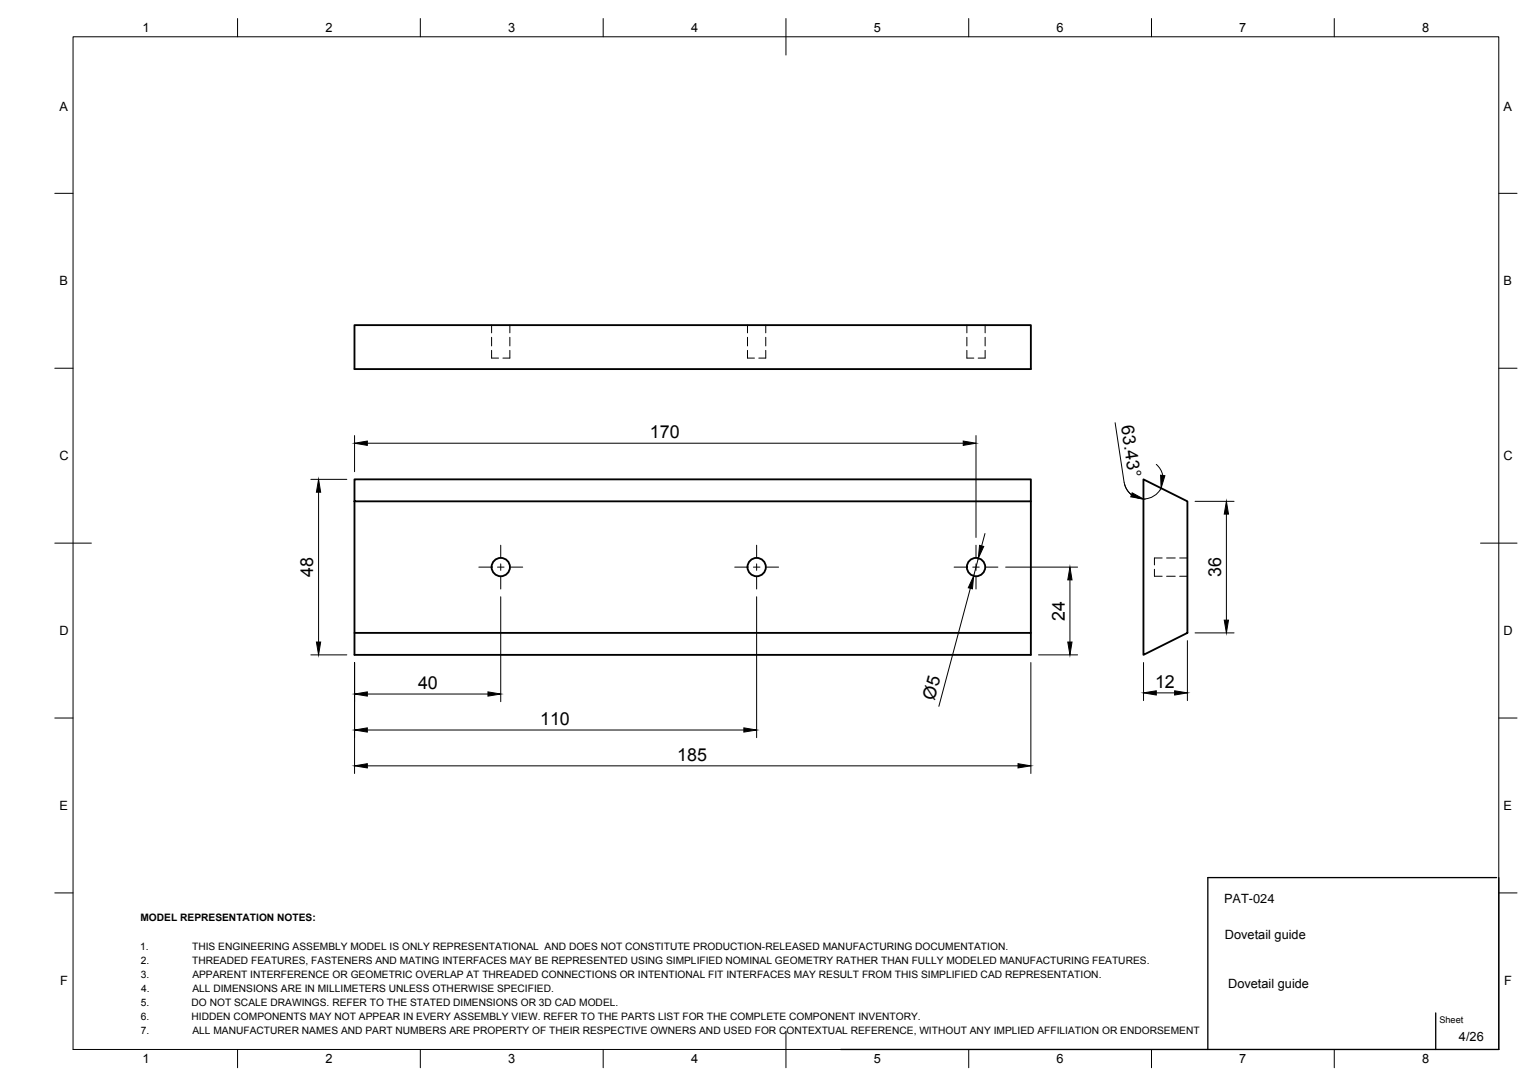
ISO-10303-21;
HEADER;
/* Generated by software containing ST-Developer
 * from STEP Tools, Inc. (www.steptools.com) 
 */

FILE_DESCRIPTION(
/* description */ ('Compact handwheel screw vise'),
/* implementation_level */ '2;1');

FILE_NAME(
/* name */ 'Dovetail guide.step',
/* time_stamp */ '2026-10-29T16:08:22-07:00',
/* author */ (''),
/* organization */ (''),
/* preprocessor_version */ 'ST-DEVELOPER v20.2',
/* originating_system */ 'Autodesk Translation Framework v15.17.0.0',
/* authorisation */ '');

FILE_SCHEMA (('AUTOMOTIVE_DESIGN { 1 0 10303 214 3 1 1 }'));
ENDSEC;

DATA;
#10=MECHANICAL_DESIGN_GEOMETRIC_PRESENTATION_REPRESENTATION('',(#645),#25074);
#589=SHAPE_REPRESENTATION_RELATIONSHIP('SRR','None',#25197,#617);
#617=ADVANCED_BREP_SHAPE_REPRESENTATION('',(#681),#25044);
#645=STYLED_ITEM('',(#25425),#681);
#681=MANIFOLD_SOLID_BREP('Body1',#8053);
#726=FACE_BOUND('',#1518,.T.);
#727=FACE_BOUND('',#1519,.T.);
#728=FACE_BOUND('',#1520,.T.);
#828=PLANE('',#8435);
#829=PLANE('',#8439);
#830=PLANE('',#8443);
#831=PLANE('',#8444);
#832=PLANE('',#8445);
#833=PLANE('',#8446);
#834=PLANE('',#8447);
#835=PLANE('',#8448);
#836=PLANE('',#8449);
#1025=FACE_OUTER_BOUND('',#1509,.T.);
#1026=FACE_OUTER_BOUND('',#1510,.T.);
#1027=FACE_OUTER_BOUND('',#1511,.T.);
#1028=FACE_OUTER_BOUND('',#1512,.T.);
#1029=FACE_OUTER_BOUND('',#1513,.T.);
#1030=FACE_OUTER_BOUND('',#1514,.T.);
#1031=FACE_OUTER_BOUND('',#1515,.T.);
#1032=FACE_OUTER_BOUND('',#1516,.T.);
#1033=FACE_OUTER_BOUND('',#1517,.T.);
#1034=FACE_OUTER_BOUND('',#1521,.T.);
#1035=FACE_OUTER_BOUND('',#1522,.T.);
#1036=FACE_OUTER_BOUND('',#1523,.T.);
#1509=EDGE_LOOP('',(#5225,#5226,#5227,#5228));
#1510=EDGE_LOOP('',(#5229));
#1511=EDGE_LOOP('',(#5230,#5231,#5232,#5233));
#1512=EDGE_LOOP('',(#5234));
#1513=EDGE_LOOP('',(#5235,#5236,#5237,#5238));
#1514=EDGE_LOOP('',(#5239));
#1515=EDGE_LOOP('',(#5240,#5241,#5242,#5243));
#1516=EDGE_LOOP('',(#5244,#5245,#5246,#5247));
#1517=EDGE_LOOP('',(#5248,#5249,#5250,#5251));
#1518=EDGE_LOOP('',(#5252));
#1519=EDGE_LOOP('',(#5253));
#1520=EDGE_LOOP('',(#5254));
#1521=EDGE_LOOP('',(#5255,#5256,#5257,#5258));
#1522=EDGE_LOOP('',(#5259,#5260,#5261,#5262));
#1523=EDGE_LOOP('',(#5263,#5264,#5265,#5266));
#2081=LINE('',#11394,#2589);
#2082=LINE('',#11401,#2590);
#2083=LINE('',#11408,#2591);
#2084=LINE('',#11414,#2592);
#2085=LINE('',#11416,#2593);
#2086=LINE('',#11418,#2594);
#2087=LINE('',#11419,#2595);
#2088=LINE('',#11422,#2596);
#2089=LINE('',#11424,#2597);
#2090=LINE('',#11425,#2598);
#2091=LINE('',#11428,#2599);
#2092=LINE('',#11430,#2600);
#2093=LINE('',#11431,#2601);
#2094=LINE('',#11433,#2602);
#2095=LINE('',#11434,#2603);
#2589=VECTOR('',#9289,0.25);
#2590=VECTOR('',#9298,0.25);
#2591=VECTOR('',#9307,0.25);
#2592=VECTOR('',#9314,1.);
#2593=VECTOR('',#9315,1.);
#2594=VECTOR('',#9316,1.);
#2595=VECTOR('',#9317,1.);
#2596=VECTOR('',#9320,1.);
#2597=VECTOR('',#9321,1.);
#2598=VECTOR('',#9322,1.);
#2599=VECTOR('',#9325,1.);
#2600=VECTOR('',#9326,1.);
#2601=VECTOR('',#9327,1.);
#2602=VECTOR('',#9330,1.);
#2603=VECTOR('',#9331,1.);
#3092=CIRCLE('',#8433,0.25);
#3093=CIRCLE('',#8434,0.25);
#3094=CIRCLE('',#8437,0.25);
#3095=CIRCLE('',#8438,0.25);
#3096=CIRCLE('',#8441,0.25);
#3097=CIRCLE('',#8442,0.25);
#3355=VERTEX_POINT('',#11391);
#3356=VERTEX_POINT('',#11393);
#3357=VERTEX_POINT('',#11398);
#3358=VERTEX_POINT('',#11400);
#3359=VERTEX_POINT('',#11405);
#3360=VERTEX_POINT('',#11407);
#3361=VERTEX_POINT('',#11412);
#3362=VERTEX_POINT('',#11413);
#3363=VERTEX_POINT('',#11415);
#3364=VERTEX_POINT('',#11417);
#3365=VERTEX_POINT('',#11421);
#3366=VERTEX_POINT('',#11423);
#3367=VERTEX_POINT('',#11427);
#3368=VERTEX_POINT('',#11429);
#4099=EDGE_CURVE('',#3355,#3355,#3092,.T.);
#4100=EDGE_CURVE('',#3355,#3356,#2081,.T.);
#4101=EDGE_CURVE('',#3356,#3356,#3093,.T.);
#4102=EDGE_CURVE('',#3357,#3357,#3094,.T.);
#4103=EDGE_CURVE('',#3357,#3358,#2082,.T.);
#4104=EDGE_CURVE('',#3358,#3358,#3095,.T.);
#4105=EDGE_CURVE('',#3359,#3359,#3096,.T.);
#4106=EDGE_CURVE('',#3359,#3360,#2083,.T.);
#4107=EDGE_CURVE('',#3360,#3360,#3097,.T.);
#4108=EDGE_CURVE('',#3361,#3362,#2084,.T.);
#4109=EDGE_CURVE('',#3362,#3363,#2085,.T.);
#4110=EDGE_CURVE('',#3364,#3363,#2086,.T.);
#4111=EDGE_CURVE('',#3361,#3364,#2087,.T.);
#4112=EDGE_CURVE('',#3365,#3361,#2088,.T.);
#4113=EDGE_CURVE('',#3366,#3364,#2089,.T.);
#4114=EDGE_CURVE('',#3365,#3366,#2090,.T.);
#4115=EDGE_CURVE('',#3367,#3365,#2091,.T.);
#4116=EDGE_CURVE('',#3368,#3366,#2092,.T.);
#4117=EDGE_CURVE('',#3367,#3368,#2093,.T.);
#4118=EDGE_CURVE('',#3362,#3367,#2094,.T.);
#4119=EDGE_CURVE('',#3363,#3368,#2095,.T.);
#5225=ORIENTED_EDGE('',*,*,#4099,.F.);
#5226=ORIENTED_EDGE('',*,*,#4100,.T.);
#5227=ORIENTED_EDGE('',*,*,#4101,.T.);
#5228=ORIENTED_EDGE('',*,*,#4100,.F.);
#5229=ORIENTED_EDGE('',*,*,#4101,.F.);
#5230=ORIENTED_EDGE('',*,*,#4102,.F.);
#5231=ORIENTED_EDGE('',*,*,#4103,.T.);
#5232=ORIENTED_EDGE('',*,*,#4104,.T.);
#5233=ORIENTED_EDGE('',*,*,#4103,.F.);
#5234=ORIENTED_EDGE('',*,*,#4104,.F.);
#5235=ORIENTED_EDGE('',*,*,#4105,.F.);
#5236=ORIENTED_EDGE('',*,*,#4106,.T.);
#5237=ORIENTED_EDGE('',*,*,#4107,.T.);
#5238=ORIENTED_EDGE('',*,*,#4106,.F.);
#5239=ORIENTED_EDGE('',*,*,#4107,.F.);
#5240=ORIENTED_EDGE('',*,*,#4108,.T.);
#5241=ORIENTED_EDGE('',*,*,#4109,.T.);
#5242=ORIENTED_EDGE('',*,*,#4110,.F.);
#5243=ORIENTED_EDGE('',*,*,#4111,.F.);
#5244=ORIENTED_EDGE('',*,*,#4112,.T.);
#5245=ORIENTED_EDGE('',*,*,#4111,.T.);
#5246=ORIENTED_EDGE('',*,*,#4113,.F.);
#5247=ORIENTED_EDGE('',*,*,#4114,.F.);
#5248=ORIENTED_EDGE('',*,*,#4115,.T.);
#5249=ORIENTED_EDGE('',*,*,#4114,.T.);
#5250=ORIENTED_EDGE('',*,*,#4116,.F.);
#5251=ORIENTED_EDGE('',*,*,#4117,.F.);
#5252=ORIENTED_EDGE('',*,*,#4099,.T.);
#5253=ORIENTED_EDGE('',*,*,#4102,.T.);
#5254=ORIENTED_EDGE('',*,*,#4105,.T.);
#5255=ORIENTED_EDGE('',*,*,#4118,.T.);
#5256=ORIENTED_EDGE('',*,*,#4117,.T.);
#5257=ORIENTED_EDGE('',*,*,#4119,.F.);
#5258=ORIENTED_EDGE('',*,*,#4109,.F.);
#5259=ORIENTED_EDGE('',*,*,#4119,.T.);
#5260=ORIENTED_EDGE('',*,*,#4116,.T.);
#5261=ORIENTED_EDGE('',*,*,#4113,.T.);
#5262=ORIENTED_EDGE('',*,*,#4110,.T.);
#5263=ORIENTED_EDGE('',*,*,#4118,.F.);
#5264=ORIENTED_EDGE('',*,*,#4108,.F.);
#5265=ORIENTED_EDGE('',*,*,#4112,.F.);
#5266=ORIENTED_EDGE('',*,*,#4115,.F.);
#7352=CYLINDRICAL_SURFACE('',#8432,0.25);
#7353=CYLINDRICAL_SURFACE('',#8436,0.25);
#7354=CYLINDRICAL_SURFACE('',#8440,0.25);
#7595=ADVANCED_FACE('',(#1025),#7352,.F.);
#7596=ADVANCED_FACE('',(#1026),#828,.F.);
#7597=ADVANCED_FACE('',(#1027),#7353,.F.);
#7598=ADVANCED_FACE('',(#1028),#829,.F.);
#7599=ADVANCED_FACE('',(#1029),#7354,.F.);
#7600=ADVANCED_FACE('',(#1030),#830,.F.);
#7601=ADVANCED_FACE('',(#1031),#831,.T.);
#7602=ADVANCED_FACE('',(#1032),#832,.T.);
#7603=ADVANCED_FACE('',(#1033,#726,#727,#728),#833,.T.);
#7604=ADVANCED_FACE('',(#1034),#834,.T.);
#7605=ADVANCED_FACE('',(#1035),#835,.T.);
#7606=ADVANCED_FACE('',(#1036),#836,.F.);
#8053=CLOSED_SHELL('',(#7595,#7596,#7597,#7598,#7599,#7600,#7601,#7602,
#7603,#7604,#7605,#7606));
#8431=AXIS2_PLACEMENT_3D('',#11389,#9283,#9284);
#8432=AXIS2_PLACEMENT_3D('',#11390,#9285,#9286);
#8433=AXIS2_PLACEMENT_3D('',#11392,#9287,#9288);
#8434=AXIS2_PLACEMENT_3D('',#11395,#9290,#9291);
#8435=AXIS2_PLACEMENT_3D('',#11396,#9292,#9293);
#8436=AXIS2_PLACEMENT_3D('',#11397,#9294,#9295);
#8437=AXIS2_PLACEMENT_3D('',#11399,#9296,#9297);
#8438=AXIS2_PLACEMENT_3D('',#11402,#9299,#9300);
#8439=AXIS2_PLACEMENT_3D('',#11403,#9301,#9302);
#8440=AXIS2_PLACEMENT_3D('',#11404,#9303,#9304);
#8441=AXIS2_PLACEMENT_3D('',#11406,#9305,#9306);
#8442=AXIS2_PLACEMENT_3D('',#11409,#9308,#9309);
#8443=AXIS2_PLACEMENT_3D('',#11410,#9310,#9311);
#8444=AXIS2_PLACEMENT_3D('',#11411,#9312,#9313);
#8445=AXIS2_PLACEMENT_3D('',#11420,#9318,#9319);
#8446=AXIS2_PLACEMENT_3D('',#11426,#9323,#9324);
#8447=AXIS2_PLACEMENT_3D('',#11432,#9328,#9329);
#8448=AXIS2_PLACEMENT_3D('',#11435,#9332,#9333);
#8449=AXIS2_PLACEMENT_3D('',#11436,#9334,#9335);
#9283=DIRECTION('axis',(0.,0.,1.));
#9284=DIRECTION('refdir',(1.,0.,0.));
#9285=DIRECTION('center_axis',(0.,0.,1.));
#9286=DIRECTION('ref_axis',(1.,0.,0.));
#9287=DIRECTION('center_axis',(0.,0.,1.));
#9288=DIRECTION('ref_axis',(1.,0.,0.));
#9289=DIRECTION('',(0.,0.,1.));
#9290=DIRECTION('center_axis',(0.,0.,1.));
#9291=DIRECTION('ref_axis',(1.,0.,0.));
#9292=DIRECTION('center_axis',(0.,0.,1.));
#9293=DIRECTION('ref_axis',(1.,0.,0.));
#9294=DIRECTION('center_axis',(0.,0.,1.));
#9295=DIRECTION('ref_axis',(1.,0.,0.));
#9296=DIRECTION('center_axis',(0.,0.,1.));
#9297=DIRECTION('ref_axis',(1.,0.,0.));
#9298=DIRECTION('',(0.,0.,1.));
#9299=DIRECTION('center_axis',(0.,0.,1.));
#9300=DIRECTION('ref_axis',(1.,0.,0.));
#9301=DIRECTION('center_axis',(0.,0.,1.));
#9302=DIRECTION('ref_axis',(1.,0.,0.));
#9303=DIRECTION('center_axis',(0.,0.,1.));
#9304=DIRECTION('ref_axis',(1.,0.,0.));
#9305=DIRECTION('center_axis',(0.,0.,1.));
#9306=DIRECTION('ref_axis',(1.,0.,0.));
#9307=DIRECTION('',(0.,0.,1.));
#9308=DIRECTION('center_axis',(0.,0.,1.));
#9309=DIRECTION('ref_axis',(1.,0.,0.));
#9310=DIRECTION('center_axis',(0.,0.,1.));
#9311=DIRECTION('ref_axis',(1.,0.,0.));
#9312=DIRECTION('center_axis',(0.,0.,1.));
#9313=DIRECTION('ref_axis',(0.,-1.,0.));
#9314=DIRECTION('',(0.,-1.,0.));
#9315=DIRECTION('',(1.,0.,0.));
#9316=DIRECTION('',(0.,-1.,0.));
#9317=DIRECTION('',(1.,0.,0.));
#9318=DIRECTION('center_axis',(0.,0.894427190999916,-0.447213595499958));
#9319=DIRECTION('ref_axis',(0.,0.447213595499958,0.894427190999916));
#9320=DIRECTION('',(0.,0.447213595499958,0.894427190999916));
#9321=DIRECTION('',(0.,0.447213595499958,0.894427190999916));
#9322=DIRECTION('',(1.,0.,0.));
#9323=DIRECTION('center_axis',(0.,0.,-1.));
#9324=DIRECTION('ref_axis',(0.,1.,0.));
#9325=DIRECTION('',(0.,1.,0.));
#9326=DIRECTION('',(0.,1.,0.));
#9327=DIRECTION('',(1.,0.,0.));
#9328=DIRECTION('center_axis',(0.,-0.894427190999916,-0.447213595499958));
#9329=DIRECTION('ref_axis',(0.,0.447213595499958,-0.894427190999916));
#9330=DIRECTION('',(0.,0.447213595499958,-0.894427190999916));
#9331=DIRECTION('',(0.,0.447213595499958,-0.894427190999916));
#9332=DIRECTION('center_axis',(1.,0.,0.));
#9333=DIRECTION('ref_axis',(0.,0.,-1.));
#9334=DIRECTION('center_axis',(1.,0.,0.));
#9335=DIRECTION('ref_axis',(0.,0.,-1.));
#11389=CARTESIAN_POINT('',(0.,0.,0.));
#11390=CARTESIAN_POINT('Origin',(5.,0.,1.1));
#11391=CARTESIAN_POINT('',(4.75,-3.06161699786838E-17,1.2));
#11392=CARTESIAN_POINT('Origin',(5.,0.,1.2));
#11393=CARTESIAN_POINT('',(4.75,-3.06161699786838E-17,2.1));
#11394=CARTESIAN_POINT('',(4.75,-3.06161699786838E-17,1.1));
#11395=CARTESIAN_POINT('Origin',(5.,0.,2.1));
#11396=CARTESIAN_POINT('Origin',(5.,0.,2.1));
#11397=CARTESIAN_POINT('Origin',(11.,0.,1.1));
#11398=CARTESIAN_POINT('',(10.75,-3.06161699786838E-17,1.2));
#11399=CARTESIAN_POINT('Origin',(11.,0.,1.2));
#11400=CARTESIAN_POINT('',(10.75,-3.06161699786838E-17,2.1));
#11401=CARTESIAN_POINT('',(10.75,-3.06161699786838E-17,1.1));
#11402=CARTESIAN_POINT('Origin',(11.,0.,2.1));
#11403=CARTESIAN_POINT('Origin',(11.,0.,2.1));
#11404=CARTESIAN_POINT('Origin',(18.,0.,1.1));
#11405=CARTESIAN_POINT('',(17.75,-3.06161699786838E-17,1.2));
#11406=CARTESIAN_POINT('Origin',(18.,0.,1.2));
#11407=CARTESIAN_POINT('',(17.75,-3.06161699786838E-17,2.1));
#11408=CARTESIAN_POINT('',(17.75,-3.06161699786838E-17,1.1));
#11409=CARTESIAN_POINT('Origin',(18.,0.,2.1));
#11410=CARTESIAN_POINT('Origin',(18.,0.,2.1));
#11411=CARTESIAN_POINT('Origin',(3.5,2.4,2.4));
#11412=CARTESIAN_POINT('',(3.5,2.4,2.4));
#11413=CARTESIAN_POINT('',(3.5,-2.4,2.4));
#11414=CARTESIAN_POINT('',(3.5,2.4,2.4));
#11415=CARTESIAN_POINT('',(22.,-2.4,2.4));
#11416=CARTESIAN_POINT('',(3.5,-2.4,2.4));
#11417=CARTESIAN_POINT('',(22.,2.4,2.4));
#11418=CARTESIAN_POINT('',(22.,2.4,2.4));
#11419=CARTESIAN_POINT('',(3.5,2.4,2.4));
#11420=CARTESIAN_POINT('Origin',(3.5,1.8,1.2));
#11421=CARTESIAN_POINT('',(3.5,1.8,1.2));
#11422=CARTESIAN_POINT('',(3.5,1.8,1.2));
#11423=CARTESIAN_POINT('',(22.,1.8,1.2));
#11424=CARTESIAN_POINT('',(22.,1.8,1.2));
#11425=CARTESIAN_POINT('',(3.5,1.8,1.2));
#11426=CARTESIAN_POINT('Origin',(3.5,-1.8,1.2));
#11427=CARTESIAN_POINT('',(3.5,-1.8,1.2));
#11428=CARTESIAN_POINT('',(3.5,-1.8,1.2));
#11429=CARTESIAN_POINT('',(22.,-1.8,1.2));
#11430=CARTESIAN_POINT('',(22.,-1.8,1.2));
#11431=CARTESIAN_POINT('',(3.5,-1.8,1.2));
#11432=CARTESIAN_POINT('Origin',(3.5,-2.4,2.4));
#11433=CARTESIAN_POINT('',(3.5,-2.4,2.4));
#11434=CARTESIAN_POINT('',(22.,-2.4,2.4));
#11435=CARTESIAN_POINT('Origin',(22.,0.,1.8));
#11436=CARTESIAN_POINT('Origin',(3.5,0.,1.8));
#25010=UNCERTAINTY_MEASURE_WITH_UNIT(LENGTH_MEASURE(0.001),#25075,
'DISTANCE_ACCURACY_VALUE',
'Maximum model space distance between geometric entities at asserted c
onnectivities');
#25040=UNCERTAINTY_MEASURE_WITH_UNIT(LENGTH_MEASURE(0.001),#25075,
'DISTANCE_ACCURACY_VALUE',
'Maximum model space distance between geometric entities at asserted c
onnectivities');
#25044=(
GEOMETRIC_REPRESENTATION_CONTEXT(3)
GLOBAL_UNCERTAINTY_ASSIGNED_CONTEXT((#25010))
GLOBAL_UNIT_ASSIGNED_CONTEXT((#25075,#25077,#25078))
REPRESENTATION_CONTEXT('','3D')
);
#25074=(
GEOMETRIC_REPRESENTATION_CONTEXT(3)
GLOBAL_UNCERTAINTY_ASSIGNED_CONTEXT((#25040))
GLOBAL_UNIT_ASSIGNED_CONTEXT((#25075,#25077,#25078))
REPRESENTATION_CONTEXT('','3D')
);
#25075=(
LENGTH_UNIT()
NAMED_UNIT(*)
SI_UNIT(.CENTI.,.METRE.)
);
#25077=(
NAMED_UNIT(*)
PLANE_ANGLE_UNIT()
SI_UNIT($,.RADIAN.)
);
#25078=(
NAMED_UNIT(*)
SI_UNIT($,.STERADIAN.)
SOLID_ANGLE_UNIT()
);
#25082=SHAPE_DEFINITION_REPRESENTATION(#25115,#25197);
#25115=PRODUCT_DEFINITION_SHAPE('',$,#25231);
#25197=SHAPE_REPRESENTATION('',(#8431),#25044);
#25227=PRODUCT_DEFINITION_CONTEXT('part definition',#25328,'design');
#25231=PRODUCT_DEFINITION('Dovetail guide','Dovetail guide',#25264,#25227);
#25264=PRODUCT_DEFINITION_FORMATION('',$,#25333);
#25328=APPLICATION_CONTEXT(
'Core Data for Automotive Mechanical Design Process');
#25329=PRODUCT_CONTEXT('part definition',#25328,'mechanical');
#25333=PRODUCT('Dovetail guide','Dovetail guide','Dovetail guide',(#25329));
#25419=COLOUR_RGB('Light Blue',0.38,0.62,0.78);
#25420=FILL_AREA_STYLE_COLOUR('',#25419);
#25421=FILL_AREA_STYLE('',(#25420));
#25422=SURFACE_STYLE_FILL_AREA(#25421);
#25423=SURFACE_SIDE_STYLE('',(#25422));
#25424=SURFACE_STYLE_USAGE(.BOTH.,#25423);
#25425=PRESENTATION_STYLE_ASSIGNMENT((#25424));
ENDSEC;
END-ISO-10303-21;
